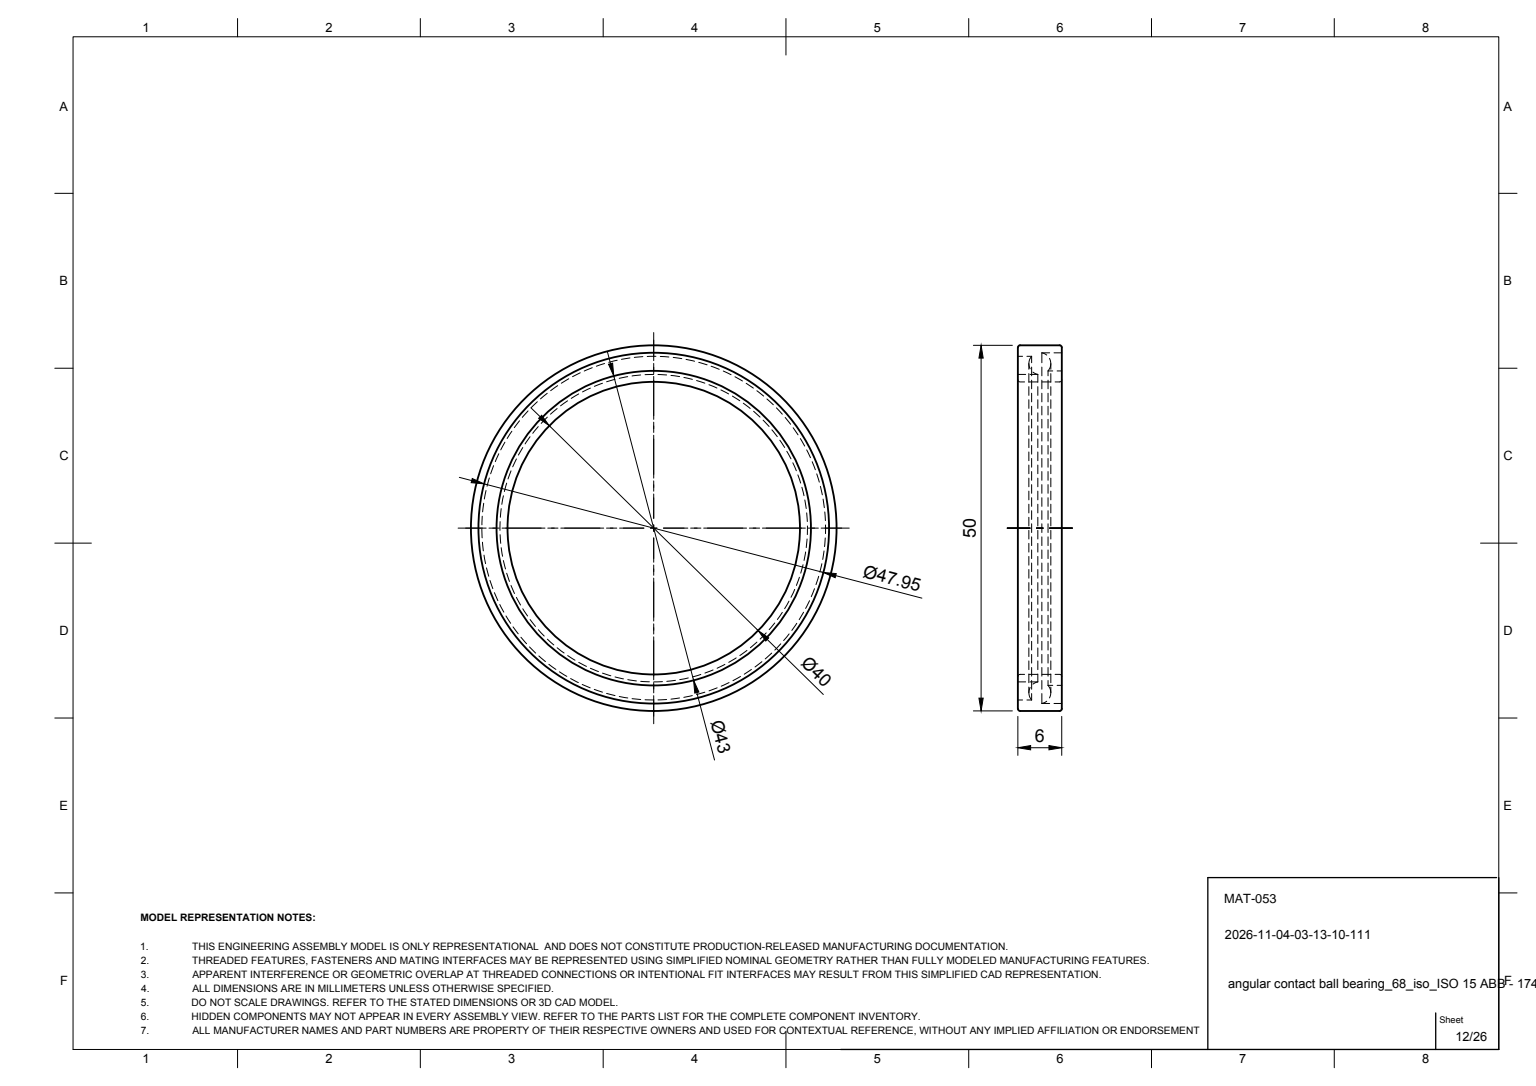
ISO-10303-21;
HEADER;
FILE_DESCRIPTION (('STEP AP214'),
    '1' );
FILE_NAME ('angular contact ball bearing_68_iso_ISO 15 ABB - 1740 - 38,SI,NC,38_68.step',
    '2026-10-10T03:43:58',
    ( '' ),
    ( '' ),
    'SwSTEP 2.0',
    'SolidWorks 2026',
    '' );
FILE_SCHEMA (( 'AUTOMOTIVE_DESIGN' ));
ENDSEC;

DATA;
#280=CARTESIAN_POINT ( 'NONE',  ( -20.63749999999999574, 0.000000000000000000, 0.000000000000000000 ) ) ;
#290=CYLINDRICAL_SURFACE ( 'NONE', #39876, 21.02500000000000213 ) ;
#373=EDGE_CURVE ( 'NONE', #61321, #29458, #45223, .T. ) ;
#397=AXIS2_PLACEMENT_3D ( 'NONE', #30126, #55451, #24841 ) ;
#538=EDGE_CURVE ( 'NONE', #52559, #9895, #28349, .T. ) ;
#593=CARTESIAN_POINT ( 'NONE',  ( 3.000000000000002665, 0.000000000000000000, 0.000000000000000000 ) ) ;
#621=( GEOMETRIC_REPRESENTATION_CONTEXT ( 3 ) GLOBAL_UNCERTAINTY_ASSIGNED_CONTEXT ( ( #45151 ) ) GLOBAL_UNIT_ASSIGNED_CONTEXT ( ( #57453, #30034, #6044 ) ) REPRESENTATION_CONTEXT ( 'NONE', 'WORKASPACE' ) );
#645=DIRECTION ( 'NONE',  ( -1.000000000000000000, -0.000000000000000000, -0.000000000000000000 ) ) ;
#660=AXIS2_PLACEMENT_3D ( 'NONE', #33851, #12745, #56006 ) ;
#969=CIRCLE ( 'NONE', #42531, 0.3000000000000051514 ) ;
#1025=DIRECTION ( 'NONE',  ( -0.000000000000000000, 0.000000000000000000, 1.000000000000000000 ) ) ;
#1055=EDGE_LOOP ( 'NONE', ( #53256, #11888, #11752, #31216 ) ) ;
#1105=CARTESIAN_POINT ( 'NONE',  ( -20.63749999999999929, 2.574819895207310592E-15, 21.02500000000000213 ) ) ;
#1307=EDGE_LOOP ( 'NONE', ( #35299, #10153, #10005, #63339 ) ) ;
#1323=TOROIDAL_SURFACE ( 'NONE', #20399, 22.50000000000000000, 1.500000000000000444 ) ;
#1417=AXIS2_PLACEMENT_3D ( 'NONE', #30152, #18895, #57567 ) ;
#1469=SURFACE_SIDE_STYLE ('',( #55275 ) ) ;
#1536=CARTESIAN_POINT ( 'NONE',  ( 3.000000000000006217, 0.000000000000000000, 0.000000000000000000 ) ) ;
#1545=ORIENTED_EDGE ( 'NONE', *, *, #39490, .T. ) ;
#1648=FACE_OUTER_BOUND ( 'NONE', #49556, .T. ) ;
#1676=AXIS2_PLACEMENT_3D ( 'NONE', #6098, #53928, #48643 ) ;
#1879=CIRCLE ( 'NONE', #29940, 1.500000000000001332 ) ;
#1883=DIRECTION ( 'NONE',  ( 0.000000000000000000, 0.000000000000000000, -1.000000000000000000 ) ) ;
#1943=CARTESIAN_POINT ( 'NONE',  ( -0.2727178028659107967, 2.936090700955778964E-15, -23.97499999999999787 ) ) ;
#1945=ORIENTED_EDGE ( 'NONE', *, *, #538, .F. ) ;
#2038=CIRCLE ( 'NONE', #53667, 25.00000000000000355 ) ;
#2107=ORIENTED_EDGE ( 'NONE', *, *, #62169, .F. ) ;
#2116=DIRECTION ( 'NONE',  ( 1.000000000000000000, 0.000000000000000000, 0.000000000000000000 ) ) ;
#2288=DIRECTION ( 'NONE',  ( -0.000000000000000000, 0.000000000000000000, 1.000000000000000000 ) ) ;
#2314=ORIENTED_EDGE ( 'NONE', *, *, #36138, .T. ) ;
#2373=DIRECTION ( 'NONE',  ( 1.000000000000000000, 0.000000000000000000, 0.000000000000000000 ) ) ;
#2396=MECHANICAL_DESIGN_GEOMETRIC_PRESENTATION_REPRESENTATION('',(#32715),#59658);
#2447=CYLINDRICAL_SURFACE ( 'NONE', #33618, 25.00000000000000711 ) ;
#2492=DIRECTION ( 'NONE',  ( 0.000000000000000000, -1.000000000000000000, 0.000000000000000000 ) ) ;
#2692=CARTESIAN_POINT ( 'NONE',  ( 2.699999999999990408, 0.000000000000000000, 0.000000000000000000 ) ) ;
#2799=ADVANCED_FACE ( 'NONE', ( #20237 ), #8332, .T. ) ;
#2890=LINE ( 'NONE', #34569, #25833 ) ;
#2981=EDGE_LOOP ( 'NONE', ( #13147, #27199, #10225, #40250 ) ) ;
#3058=EDGE_CURVE ( 'NONE', #60812, #57773, #58704, .T. ) ;
#3118=CARTESIAN_POINT ( 'NONE',  ( 2.999999999999992450, 0.000000000000000000, 0.000000000000000000 ) ) ;
#3137=DIRECTION ( 'NONE',  ( 1.000000000000000000, 0.000000000000000000, 0.000000000000000000 ) ) ;
#3249=EDGE_LOOP ( 'NONE', ( #58804, #53989, #66441, #9980 ) ) ;
#3441=DIRECTION ( 'NONE',  ( 0.000000000000000000, 0.000000000000000000, -1.000000000000000000 ) ) ;
#3503=CIRCLE ( 'NONE', #56271, 24.69999999999999929 ) ;
#3556=DIRECTION ( 'NONE',  ( 1.000000000000000000, 0.000000000000000000, 0.000000000000000000 ) ) ;
#3565=DIRECTION ( 'NONE',  ( -1.000000000000000000, -0.000000000000000000, -0.000000000000000000 ) ) ;
#3692=AXIS2_PLACEMENT_3D ( 'NONE', #33582, #55008, #6830 ) ;
#3738=ORIENTED_EDGE ( 'NONE', *, *, #14434, .T. ) ;
#3880=EDGE_CURVE ( 'NONE', #19652, #60812, #44141, .T. ) ;
#4000=AXIS2_PLACEMENT_3D ( 'NONE', #32142, #21921, #69063 ) ;
#4007=CYLINDRICAL_SURFACE ( 'NONE', #6388, 23.50000000000000000 ) ;
#4031=AXIS2_PLACEMENT_3D ( 'NONE', #27744, #49185, #1025 ) ;
#4149=CIRCLE ( 'NONE', #55822, 1.500000000000001332 ) ;
#4152=ADVANCED_FACE ( 'NONE', ( #15588, #58822 ), #37037, .T. ) ;
#4194=ORIENTED_EDGE ( 'NONE', *, *, #40811, .F. ) ;
#4257=VERTEX_POINT ( 'NONE', #31338 ) ;
#4325=DIRECTION ( 'NONE',  ( 1.000000000000000000, 0.000000000000000000, 0.000000000000000000 ) ) ;
#4352=FACE_OUTER_BOUND ( 'NONE', #11897, .T. ) ;
#4484=EDGE_LOOP ( 'NONE', ( #2107, #34781, #40469, #13611 ) ) ;
#4509=AXIS2_PLACEMENT_3D ( 'NONE', #52504, #4325, #66976 ) ;
#4534=CARTESIAN_POINT ( 'NONE',  ( 2.699999999999990408, 2.467663300281916154E-15, 19.99999999999998934 ) ) ;
#4593=PRODUCT_DEFINITION_SHAPE ( 'NONE', 'NONE',  #56848 ) ;
#4670=DIRECTION ( 'NONE',  ( 0.000000000000000000, 0.000000000000000000, -1.000000000000000000 ) ) ;
#4680=CARTESIAN_POINT ( 'NONE',  ( -2.699999999999990408, 0.000000000000000000, 0.000000000000000000 ) ) ;
#4739=AXIS2_PLACEMENT_3D ( 'NONE', #280, #64310, #58676 ) ;
#4831=VECTOR ( 'NONE', #25004, 1000.000000000000000 ) ;
#5355=EDGE_LOOP ( 'NONE', ( #29578, #35095, #48562, #52524 ) ) ;
#5423=ORIENTED_EDGE ( 'NONE', *, *, #38504, .T. ) ;
#5446=DIRECTION ( 'NONE',  ( 1.000000000000000000, 0.000000000000000000, 0.000000000000000000 ) ) ;
#5645=EDGE_CURVE ( 'NONE', #52559, #6514, #31915, .T. ) ;
#5676=AXIS2_PLACEMENT_3D ( 'NONE', #13153, #67320, #40560 ) ;
#5689=PRESENTATION_STYLE_ASSIGNMENT (( #49641 ) ) ;
#5737=DIRECTION ( 'NONE',  ( 0.000000000000000000, 0.000000000000000000, -1.000000000000000000 ) ) ;
#6044=( NAMED_UNIT ( * ) SI_UNIT ( $, .STERADIAN. ) SOLID_ANGLE_UNIT ( ) );
#6069=TOROIDAL_SURFACE ( 'NONE', #61121, 20.30000000000000071, 0.3000000000000062061 ) ;
#6074=CIRCLE ( 'NONE', #45411, 0.3000000000000051514 ) ;
#6098=CARTESIAN_POINT ( 'NONE',  ( -2.699999999999990408, 0.000000000000000000, 0.000000000000000000 ) ) ;
#6152=ORIENTED_EDGE ( 'NONE', *, *, #29172, .T. ) ;
#6170=AXIS2_PLACEMENT_3D ( 'NONE', #8294, #46253, #41679 ) ;
#6245=DIRECTION ( 'NONE',  ( 0.000000000000000000, 1.000000000000000000, -1.224646799147353207E-16 ) ) ;
#6250=DIRECTION ( 'NONE',  ( 0.000000000000000000, 0.000000000000000000, -1.000000000000000000 ) ) ;
#6260=CARTESIAN_POINT ( 'NONE',  ( 0.2727178028659107412, 0.000000000000000000, 0.000000000000000000 ) ) ;
#6278=DIRECTION ( 'NONE',  ( 0.000000000000000000, 1.000000000000000000, -1.224646799147353207E-16 ) ) ;
#6294=FACE_OUTER_BOUND ( 'NONE', #48770, .T. ) ;
#6341=EDGE_CURVE ( 'NONE', #42528, #57773, #66837, .T. ) ;
#6372=DIRECTION ( 'NONE',  ( 1.000000000000000000, 0.000000000000000000, 0.000000000000000000 ) ) ;
#6388=AXIS2_PLACEMENT_3D ( 'NONE', #14557, #51162, #19139 ) ;
#6392=CIRCLE ( 'NONE', #41248, 23.97499999999999787 ) ;
#6514=VERTEX_POINT ( 'NONE', #4534 ) ;
#6524=CARTESIAN_POINT ( 'NONE',  ( 0.2727178028659107412, 0.000000000000000000, 21.02500000000000213 ) ) ;
#6527=EDGE_LOOP ( 'NONE', ( #17045, #8583, #48179, #6821 ) ) ;
#6821=ORIENTED_EDGE ( 'NONE', *, *, #45518, .F. ) ;
#6830=DIRECTION ( 'NONE',  ( 0.000000000000000000, -1.224646799147351975E-16, 1.000000000000000000 ) ) ;
#6953=DIRECTION ( 'NONE',  ( -1.000000000000000000, -0.000000000000000000, -0.000000000000000000 ) ) ;
#7109=AXIS2_PLACEMENT_3D ( 'NONE', #17385, #52177, #56771 ) ;
#7160=ORIENTED_EDGE ( 'NONE', *, *, #39490, .F. ) ;
#7202=DIRECTION ( 'NONE',  ( 1.000000000000000000, 0.000000000000000000, 0.000000000000000000 ) ) ;
#7301=CIRCLE ( 'NONE', #6170, 23.97499999999999787 ) ;
#7431=DIRECTION ( 'NONE',  ( 0.000000000000000000, 0.000000000000000000, -1.000000000000000000 ) ) ;
#7736=DIRECTION ( 'NONE',  ( 0.000000000000000000, 0.000000000000000000, 1.000000000000000000 ) ) ;
#7907=ORIENTED_EDGE ( 'NONE', *, *, #42027, .T. ) ;
#7941=ORIENTED_EDGE ( 'NONE', *, *, #41756, .F. ) ;
#8069=LINE ( 'NONE', #52019, #34673 ) ;
#8081=ORIENTED_EDGE ( 'NONE', *, *, #9301, .F. ) ;
#8105=CIRCLE ( 'NONE', #49656, 0.3000000000000051514 ) ;
#8217=FACE_OUTER_BOUND ( 'NONE', #67323, .T. ) ;
#8282=ORIENTED_EDGE ( 'NONE', *, *, #373, .T. ) ;
#8294=CARTESIAN_POINT ( 'NONE',  ( -3.000000000000006217, 0.000000000000000000, 0.000000000000000000 ) ) ;
#8299=CARTESIAN_POINT ( 'NONE',  ( 3.000000000000002665, 0.000000000000000000, 0.000000000000000000 ) ) ;
#8307=FACE_OUTER_BOUND ( 'NONE', #58252, .T. ) ;
#8319=DIRECTION ( 'NONE',  ( 1.000000000000000000, 0.000000000000000000, 0.000000000000000000 ) ) ;
#8332=TOROIDAL_SURFACE ( 'NONE', #38593, 22.50000000000000000, 1.500000000000000444 ) ;
#8508=CIRCLE ( 'NONE', #25338, 23.50000000000000000 ) ;
#8570=FACE_BOUND ( 'NONE', #68279, .T. ) ;
#8583=ORIENTED_EDGE ( 'NONE', *, *, #38351, .T. ) ;
#8602=FACE_OUTER_BOUND ( 'NONE', #58165, .T. ) ;
#8641=FACE_OUTER_BOUND ( 'NONE', #30628, .T. ) ;
#8658=DIRECTION ( 'NONE',  ( 1.000000000000000000, 0.000000000000000000, 0.000000000000000000 ) ) ;
#8689=ORIENTED_EDGE ( 'NONE', *, *, #38093, .T. ) ;
#8731=CARTESIAN_POINT ( 'NONE',  ( 0.000000000000000000, 0.000000000000000000, 22.50000000000000000 ) ) ;
#8749=DIRECTION ( 'NONE',  ( 0.000000000000000000, 0.000000000000000000, -1.000000000000000000 ) ) ;
#8764=CARTESIAN_POINT ( 'NONE',  ( 2.699999999999990408, 0.000000000000000000, -20.30000000000000071 ) ) ;
#8768=EDGE_CURVE ( 'NONE', #9895, #52559, #26535, .T. ) ;
#8902=ORIENTED_EDGE ( 'NONE', *, *, #22144, .F. ) ;
#8954=DIRECTION ( 'NONE',  ( 1.000000000000000000, 0.000000000000000000, 0.000000000000000000 ) ) ;
#8961=EDGE_CURVE ( 'NONE', #25778, #4257, #37775, .T. ) ;
#8982=DIRECTION ( 'NONE',  ( 0.000000000000000000, 0.000000000000000000, -1.000000000000000000 ) ) ;
#8995=DIRECTION ( 'NONE',  ( 0.000000000000000000, 0.000000000000000000, -1.000000000000000000 ) ) ;
#9009=EDGE_CURVE ( 'NONE', #33511, #39615, #42211, .T. ) ;
#9167=ORIENTED_EDGE ( 'NONE', *, *, #64153, .T. ) ;
#9281=CARTESIAN_POINT ( 'NONE',  ( -2.999999999999990674, 21.50000000000000000, 0.000000000000000000 ) ) ;
#9301=EDGE_CURVE ( 'NONE', #61321, #61115, #4149, .T. ) ;
#9888=ORIENTED_EDGE ( 'NONE', *, *, #67535, .T. ) ;
#9895=VERTEX_POINT ( 'NONE', #49076 ) ;
#9905=EDGE_LOOP ( 'NONE', ( #64861, #51171, #32704, #4194 ) ) ;
#9922=CARTESIAN_POINT ( 'NONE',  ( -3.000000000000002665, 0.000000000000000000, 0.000000000000000000 ) ) ;
#9980=ORIENTED_EDGE ( 'NONE', *, *, #39856, .F. ) ;
#10005=ORIENTED_EDGE ( 'NONE', *, *, #45518, .T. ) ;
#10153=ORIENTED_EDGE ( 'NONE', *, *, #15775, .T. ) ;
#10169=AXIS2_PLACEMENT_3D ( 'NONE', #18519, #39968, #29417 ) ;
#10225=ORIENTED_EDGE ( 'NONE', *, *, #65595, .T. ) ;
#10277=FILL_AREA_STYLE ('',( #48241 ) ) ;
#10671=FACE_OUTER_BOUND ( 'NONE', #1307, .T. ) ;
#10835=CARTESIAN_POINT ( 'NONE',  ( -0.2727178028659107412, 0.000000000000000000, 0.000000000000000000 ) ) ;
#10895=VECTOR ( 'NONE', #8954, 1000.000000000000000 ) ;
#10939=CARTESIAN_POINT ( 'NONE',  ( 2.700000000000004619, 0.000000000000000000, -24.69999999999999929 ) ) ;
#11062=DIRECTION ( 'NONE',  ( 0.000000000000000000, 0.000000000000000000, -1.000000000000000000 ) ) ;
#11493=CARTESIAN_POINT ( 'NONE',  ( -3.000000000000002665, 0.000000000000000000, -24.69999999999999929 ) ) ;
#11592=CARTESIAN_POINT ( 'NONE',  ( -2.699999999999990408, 0.000000000000000000, 0.000000000000000000 ) ) ;
#11700=EDGE_LOOP ( 'NONE', ( #28380, #69331, #41144, #54488 ) ) ;
#11752=ORIENTED_EDGE ( 'NONE', *, *, #36138, .F. ) ;
#11888=ORIENTED_EDGE ( 'NONE', *, *, #36705, .T. ) ;
#11897=EDGE_LOOP ( 'NONE', ( #34288, #67277, #15013, #55475 ) ) ;
#11898=AXIS2_PLACEMENT_3D ( 'NONE', #593, #21349, #64613 ) ;
#12131=CARTESIAN_POINT ( 'NONE',  ( -20.63749999999999574, 0.000000000000000000, 0.000000000000000000 ) ) ;
#12172=CYLINDRICAL_SURFACE ( 'NONE', #65307, 23.97499999999999787 ) ;
#12227=EDGE_CURVE ( 'NONE', #27706, #49790, #6392, .T. ) ;
#12368=ORIENTED_EDGE ( 'NONE', *, *, #23031, .T. ) ;
#12612=LINE ( 'NONE', #24216, #42663 ) ;
#12629=AXIS2_PLACEMENT_3D ( 'NONE', #11592, #33073, #54500 ) ;
#12745=DIRECTION ( 'NONE',  ( 1.000000000000000000, 0.000000000000000000, 0.000000000000000000 ) ) ;
#13006=ORIENTED_EDGE ( 'NONE', *, *, #22230, .T. ) ;
#13147=ORIENTED_EDGE ( 'NONE', *, *, #67535, .F. ) ;
#13153=CARTESIAN_POINT ( 'NONE',  ( -2.999999999999992450, 0.000000000000000000, 0.000000000000000000 ) ) ;
#13239=ORIENTED_EDGE ( 'NONE', *, *, #538, .T. ) ;
#13285=CARTESIAN_POINT ( 'NONE',  ( -2.999999999999994227, 2.486033002269127373E-15, 20.30000000000000071 ) ) ;
#13313=DIRECTION ( 'NONE',  ( 0.000000000000000000, -1.000000000000000000, 0.000000000000000000 ) ) ;
#13420=DIRECTION ( 'NONE',  ( 0.000000000000000000, 0.000000000000000000, -1.000000000000000000 ) ) ;
#13611=ORIENTED_EDGE ( 'NONE', *, *, #42027, .F. ) ;
#13832=PLANE ( 'NONE',  #4509 ) ;
#13977=EDGE_CURVE ( 'NONE', #25778, #55030, #12612, .T. ) ;
#14023=DIRECTION ( 'NONE',  ( 0.000000000000000000, 0.000000000000000000, -1.000000000000000000 ) ) ;
#14189=EDGE_LOOP ( 'NONE', ( #68269, #54237, #67546, #12368 ) ) ;
#14234=CARTESIAN_POINT ( 'NONE',  ( -20.63749999999999929, 0.000000000000000000, 0.000000000000000000 ) ) ;
#14434=EDGE_CURVE ( 'NONE', #51018, #67247, #22479, .T. ) ;
#14557=CARTESIAN_POINT ( 'NONE',  ( -20.63749999999999574, 0.000000000000000000, 0.000000000000000000 ) ) ;
#14649=FACE_OUTER_BOUND ( 'NONE', #6527, .T. ) ;
#14664=CARTESIAN_POINT ( 'NONE',  ( 1.118033988749894458, 0.000000000000000000, 23.50000000000000000 ) ) ;
#14748=ADVANCED_FACE ( 'NONE', ( #8217, #8570 ), #13832, .T. ) ;
#14827=AXIS2_PLACEMENT_3D ( 'NONE', #34032, #29103, #66407 ) ;
#15013=ORIENTED_EDGE ( 'NONE', *, *, #51063, .T. ) ;
#15387=EDGE_CURVE ( 'NONE', #19256, #46466, #30421, .T. ) ;
#15483=DIRECTION ( 'NONE',  ( 1.000000000000000000, 0.000000000000000000, 0.000000000000000000 ) ) ;
#15588=FACE_OUTER_BOUND ( 'NONE', #24203, .T. ) ;
#15589=CARTESIAN_POINT ( 'NONE',  ( 3.000000000000006217, 2.877919977996280320E-15, 23.50000000000000000 ) ) ;
#15676=CARTESIAN_POINT ( 'NONE',  ( -1.118033988749894458, 0.000000000000000000, -21.50000000000000000 ) ) ;
#15775=EDGE_CURVE ( 'NONE', #44335, #54364, #3503, .T. ) ;
#16011=ORIENTED_EDGE ( 'NONE', *, *, #65424, .F. ) ;
#16224=DIRECTION ( 'NONE',  ( 0.000000000000000000, 0.000000000000000000, -1.000000000000000000 ) ) ;
#16263=CARTESIAN_POINT ( 'NONE',  ( 3.000000000000003997, 24.69999999999999929, 0.000000000000000000 ) ) ;
#16286=LINE ( 'NONE', #27882, #17334 ) ;
#16318=AXIS2_PLACEMENT_3D ( 'NONE', #14234, #18814, #68051 ) ;
#16344=CARTESIAN_POINT ( 'NONE',  ( -1.118033988749894458, 2.632990618166809235E-15, 21.50000000000000000 ) ) ;
#16665=AXIS2_PLACEMENT_3D ( 'NONE', #47766, #21050, #42497 ) ;
#16734=FACE_OUTER_BOUND ( 'NONE', #46287, .T. ) ;
#16810=VECTOR ( 'NONE', #52108, 1000.000000000000000 ) ;
#16904=ORIENTED_EDGE ( 'NONE', *, *, #31935, .F. ) ;
#17034=DIRECTION ( 'NONE',  ( 1.000000000000000000, 0.000000000000000000, 0.000000000000000000 ) ) ;
#17045=ORIENTED_EDGE ( 'NONE', *, *, #61298, .T. ) ;
#17193=ORIENTED_EDGE ( 'NONE', *, *, #64153, .F. ) ;
#17319=EDGE_LOOP ( 'NONE', ( #16011, #64545, #1545, #18990 ) ) ;
#17334=VECTOR ( 'NONE', #54952, 1000.000000000000000 ) ;
#17385=CARTESIAN_POINT ( 'NONE',  ( 0.2727178028659107412, 0.000000000000000000, 0.000000000000000000 ) ) ;
#17532=DIRECTION ( 'NONE',  ( 1.000000000000000000, 0.000000000000000000, 0.000000000000000000 ) ) ;
#17543=DIRECTION ( 'NONE',  ( 1.000000000000000000, 0.000000000000000000, 0.000000000000000000 ) ) ;
#17547=PLANE ( 'NONE',  #4031 ) ;
#17567=MANIFOLD_SOLID_BREP ( 'OuterRace', #41822 ) ;
#17705=DIRECTION ( 'NONE',  ( 1.000000000000000000, 0.000000000000000000, 0.000000000000000000 ) ) ;
#17843=AXIS2_PLACEMENT_3D ( 'NONE', #23168, #60786, #23518 ) ;
#17861=VERTEX_POINT ( 'NONE', #39721 ) ;
#17880=ORIENTED_EDGE ( 'NONE', *, *, #15387, .T. ) ;
#18211=TOROIDAL_SURFACE ( 'NONE', #14827, 22.50000000000000000, 1.500000000000000444 ) ;
#18246=AXIS2_PLACEMENT_3D ( 'NONE', #29107, #2373, #23830 ) ;
#18277=CARTESIAN_POINT ( 'NONE',  ( -20.63749999999999574, 0.000000000000000000, 0.000000000000000000 ) ) ;
#18384=CIRCLE ( 'NONE', #22907, 23.97499999999999787 ) ;
#18451=ADVANCED_FACE ( 'NONE', ( #54411 ), #18211, .T. ) ;
#18519=CARTESIAN_POINT ( 'NONE',  ( -2.999999999999992450, 0.000000000000000000, 0.000000000000000000 ) ) ;
#18814=DIRECTION ( 'NONE',  ( 1.000000000000000000, 0.000000000000000000, 0.000000000000000000 ) ) ;
#18895=DIRECTION ( 'NONE',  ( 1.000000000000000000, 0.000000000000000000, 0.000000000000000000 ) ) ;
#18903=ADVANCED_FACE ( 'NONE', ( #24777, #25130 ), #46563, .T. ) ;
#18946=CARTESIAN_POINT ( 'NONE',  ( -3.000000000000006217, 0.000000000000000000, 0.000000000000000000 ) ) ;
#18974=EDGE_LOOP ( 'NONE', ( #53039, #30160, #8689, #23492 ) ) ;
#18990=ORIENTED_EDGE ( 'NONE', *, *, #41756, .T. ) ;
#19103=CIRCLE ( 'NONE', #65146, 25.00000000000000355 ) ;
#19139=DIRECTION ( 'NONE',  ( 0.000000000000000000, 0.000000000000000000, -1.000000000000000000 ) ) ;
#19240=APPLICATION_CONTEXT ( 'automotive_design' ) ;
#19256=VERTEX_POINT ( 'NONE', #13285 ) ;
#19482=ORIENTED_EDGE ( 'NONE', *, *, #21650, .F. ) ;
#19561=DIRECTION ( 'NONE',  ( 0.000000000000000000, 0.000000000000000000, -1.000000000000000000 ) ) ;
#19652=VERTEX_POINT ( 'NONE', #6524 ) ;
#19854=FACE_OUTER_BOUND ( 'NONE', #27189, .T. ) ;
#20081=ORIENTED_EDGE ( 'NONE', *, *, #29172, .F. ) ;
#20183=EDGE_LOOP ( 'NONE', ( #2314, #17880 ) ) ;
#20189=LINE ( 'NONE', #63102, #10895 ) ;
#20237=FACE_OUTER_BOUND ( 'NONE', #26458, .T. ) ;
#20353=AXIS2_PLACEMENT_3D ( 'NONE', #12131, #17034, #49392 ) ;
#20399=AXIS2_PLACEMENT_3D ( 'NONE', #68953, #3565, #29959 ) ;
#20565=DIRECTION ( 'NONE',  ( 1.000000000000000000, 0.000000000000000000, 0.000000000000000000 ) ) ;
#20645=AXIS2_PLACEMENT_3D ( 'NONE', #23971, #66903, #13420 ) ;
#21001=CIRCLE ( 'NONE', #38941, 24.69999999999999929 ) ;
#21010=EDGE_LOOP ( 'NONE', ( #22173, #19482 ) ) ;
#21050=DIRECTION ( 'NONE',  ( 1.000000000000000000, 0.000000000000000000, 0.000000000000000000 ) ) ;
#21349=DIRECTION ( 'NONE',  ( 1.000000000000000000, 0.000000000000000000, 0.000000000000000000 ) ) ;
#21574=FACE_OUTER_BOUND ( 'NONE', #11700, .T. ) ;
#21650=EDGE_CURVE ( 'NONE', #31540, #33414, #63244, .T. ) ;
#21803=CARTESIAN_POINT ( 'NONE',  ( -2.999999999999992450, 2.632990618166809235E-15, 21.50000000000000000 ) ) ;
#21921=DIRECTION ( 'NONE',  ( 1.000000000000000000, 0.000000000000000000, 0.000000000000000000 ) ) ;
#22144=EDGE_CURVE ( 'NONE', #17861, #66051, #63291, .T. ) ;
#22173=ORIENTED_EDGE ( 'NONE', *, *, #29173, .F. ) ;
#22230=EDGE_CURVE ( 'NONE', #4257, #6514, #41435, .T. ) ;
#22432=LINE ( 'NONE', #36973, #16810 ) ;
#22479=CIRCLE ( 'NONE', #35995, 24.69999999999999929 ) ;
#22853=AXIS2_PLACEMENT_3D ( 'NONE', #64535, #5446, #11062 ) ;
#22907=AXIS2_PLACEMENT_3D ( 'NONE', #33174, #60245, #45104 ) ;
#23007=AXIS2_PLACEMENT_3D ( 'NONE', #68736, #63132, #8982 ) ;
#23031=EDGE_CURVE ( 'NONE', #55030, #6514, #28543, .T. ) ;
#23168=CARTESIAN_POINT ( 'NONE',  ( 2.699999999999990408, 0.000000000000000000, 0.000000000000000000 ) ) ;
#23260=CARTESIAN_POINT ( 'NONE',  ( -2.700000000000004619, 0.000000000000000000, -24.69999999999999929 ) ) ;
#23340=ORIENTED_EDGE ( 'NONE', *, *, #29173, .T. ) ;
#23492=ORIENTED_EDGE ( 'NONE', *, *, #45920, .F. ) ;
#23518=DIRECTION ( 'NONE',  ( 0.000000000000000000, 0.000000000000000000, -1.000000000000000000 ) ) ;
#23576=EDGE_CURVE ( 'NONE', #31797, #67247, #6074, .T. ) ;
#23614=LINE ( 'NONE', #34528, #4831 ) ;
#23830=DIRECTION ( 'NONE',  ( 0.000000000000000000, 0.000000000000000000, -1.000000000000000000 ) ) ;
#23960=ADVANCED_FACE ( 'NONE', ( #1648 ), #40996, .T. ) ;
#23971=CARTESIAN_POINT ( 'NONE',  ( 2.699999999999990408, 0.000000000000000000, 0.000000000000000000 ) ) ;
#23978=AXIS2_PLACEMENT_3D ( 'NONE', #46257, #61744, #25523 ) ;
#24203=EDGE_LOOP ( 'NONE', ( #51317, #3738 ) ) ;
#24216=CARTESIAN_POINT ( 'NONE',  ( -20.63749999999999929, 0.000000000000000000, -19.99999999999999289 ) ) ;
#24261=DIRECTION ( 'NONE',  ( 0.000000000000000000, 0.000000000000000000, -1.000000000000000000 ) ) ;
#24277=ORIENTED_EDGE ( 'NONE', *, *, #15775, .F. ) ;
#24286=CARTESIAN_POINT ( 'NONE',  ( 0.000000000000000000, 2.755455298081544778E-15, -22.50000000000000000 ) ) ;
#24770=DIRECTION ( 'NONE',  ( 0.000000000000000000, 0.000000000000000000, -1.000000000000000000 ) ) ;
#24777=FACE_BOUND ( 'NONE', #20183, .T. ) ;
#24841=DIRECTION ( 'NONE',  ( 0.000000000000000000, 0.000000000000000000, -1.000000000000000000 ) ) ;
#24845=FACE_OUTER_BOUND ( 'NONE', #3249, .T. ) ;
#24885=CIRCLE ( 'NONE', #27067, 0.3000000000000051514 ) ;
#24957=CARTESIAN_POINT ( 'NONE',  ( -3.000000000000006217, 2.936090700955778569E-15, 23.97499999999999787 ) ) ;
#25004=DIRECTION ( 'NONE',  ( 1.000000000000000000, 0.000000000000000000, 0.000000000000000000 ) ) ;
#25130=FACE_OUTER_BOUND ( 'NONE', #21010, .T. ) ;
#25190=ADVANCED_FACE ( 'NONE', ( #4352 ), #60157, .T. ) ;
#25281=CARTESIAN_POINT ( 'NONE',  ( -2.700000000000004619, 0.000000000000000000, -25.00000000000000711 ) ) ;
#25338=AXIS2_PLACEMENT_3D ( 'NONE', #1536, #44081, #33566 ) ;
#25450=ORIENTED_EDGE ( 'NONE', *, *, #49938, .F. ) ;
#25456=UNCERTAINTY_MEASURE_WITH_UNIT (LENGTH_MEASURE( 1.000000000000000082E-05 ), #48934, 'distance_accuracy_value', 'NONE');
#25517=ADVANCED_FACE ( 'NONE', ( #55292 ), #55642, .T. ) ;
#25523=DIRECTION ( 'NONE',  ( 0.000000000000000000, 0.000000000000000000, -1.000000000000000000 ) ) ;
#25778=VERTEX_POINT ( 'NONE', #59093 ) ;
#25833=VECTOR ( 'NONE', #61281, 1000.000000000000000 ) ;
#25907=DIRECTION ( 'NONE',  ( 0.000000000000000000, 1.224646799147357891E-16, 1.000000000000000000 ) ) ;
#25930=EDGE_LOOP ( 'NONE', ( #58701, #62122 ) ) ;
#26146=DIRECTION ( 'NONE',  ( 1.000000000000000000, 0.000000000000000000, 0.000000000000000000 ) ) ;
#26234=VECTOR ( 'NONE', #51646, 1000.000000000000000 ) ;
#26458=EDGE_LOOP ( 'NONE', ( #42578, #31480, #34661, #36762 ) ) ;
#26510=PRODUCT ( 'angular contact ball bearing_68_iso_ISO 15 ABB - 1740 - 38,SI,NC,38_68', 'angular contact ball bearing_68_iso_ISO 15 ABB - 1740 - 38,SI,NC,38_68', '', ( #36097 ) ) ;
#26535=CIRCLE ( 'NONE', #42303, 20.30000000000000071 ) ;
#26670=DIRECTION ( 'NONE',  ( 0.000000000000000000, 0.000000000000000000, -1.000000000000000000 ) ) ;
#27067=AXIS2_PLACEMENT_3D ( 'NONE', #61611, #38772, #60565 ) ;
#27077=AXIS2_PLACEMENT_3D ( 'NONE', #65906, #17705, #1883 ) ;
#27133=CARTESIAN_POINT ( 'NONE',  ( -20.63749999999999574, 0.000000000000000000, -23.50000000000000000 ) ) ;
#27150=EDGE_CURVE ( 'NONE', #49790, #27706, #7301, .T. ) ;
#27189=EDGE_LOOP ( 'NONE', ( #61034, #13006, #9167, #32258 ) ) ;
#27199=ORIENTED_EDGE ( 'NONE', *, *, #67117, .F. ) ;
#27347=CARTESIAN_POINT ( 'NONE',  ( -2.700000000000004619, 3.024877593893962577E-15, 24.69999999999999929 ) ) ;
#27397=EDGE_CURVE ( 'NONE', #60665, #30714, #8508, .T. ) ;
#27450=TOROIDAL_SURFACE ( 'NONE', #51081, 22.50000000000000000, 1.500000000000000444 ) ;
#27706=VERTEX_POINT ( 'NONE', #40473 ) ;
#27744=CARTESIAN_POINT ( 'NONE',  ( -3.000000000000003997, 23.97499999999999787, 0.000000000000000000 ) ) ;
#27882=CARTESIAN_POINT ( 'NONE',  ( -20.63749999999999929, 0.000000000000000000, -21.50000000000000000 ) ) ;
#27951=CYLINDRICAL_SURFACE ( 'NONE', #20353, 23.97499999999999787 ) ;
#28025=ADVANCED_FACE ( 'NONE', ( #54462, #6294 ), #17547, .T. ) ;
#28105=DIRECTION ( 'NONE',  ( 1.000000000000000000, 0.000000000000000000, 0.000000000000000000 ) ) ;
#28349=CIRCLE ( 'NONE', #29461, 20.30000000000000071 ) ;
#28380=ORIENTED_EDGE ( 'NONE', *, *, #34961, .T. ) ;
#28417=EDGE_CURVE ( 'NONE', #67247, #51018, #69191, .T. ) ;
#28479=TOROIDAL_SURFACE ( 'NONE', #397, 24.69999999999999929, 0.3000000000000035971 ) ;
#28543=CIRCLE ( 'NONE', #20645, 19.99999999999998934 ) ;
#28562=CARTESIAN_POINT ( 'NONE',  ( 3.000000000000006217, 0.000000000000000000, 0.000000000000000000 ) ) ;
#28662=DIRECTION ( 'NONE',  ( 0.000000000000000000, 0.000000000000000000, -1.000000000000000000 ) ) ;
#28700=TOROIDAL_SURFACE ( 'NONE', #4000, 24.69999999999999929, 0.3000000000000035971 ) ;
#28962=CARTESIAN_POINT ( 'NONE',  ( 2.700000000000004619, 0.000000000000000000, 0.000000000000000000 ) ) ;
#29103=DIRECTION ( 'NONE',  ( -1.000000000000000000, -0.000000000000000000, -0.000000000000000000 ) ) ;
#29107=CARTESIAN_POINT ( 'NONE',  ( -2.700000000000004619, 0.000000000000000000, 0.000000000000000000 ) ) ;
#29172=EDGE_CURVE ( 'NONE', #9895, #55030, #45658, .T. ) ;
#29173=EDGE_CURVE ( 'NONE', #33414, #31540, #47897, .T. ) ;
#29206=DIRECTION ( 'NONE',  ( -0.000000000000000000, 1.000000000000000000, 1.224646799147353207E-16 ) ) ;
#29417=DIRECTION ( 'NONE',  ( 0.000000000000000000, 0.000000000000000000, -1.000000000000000000 ) ) ;
#29458=VERTEX_POINT ( 'NONE', #43503 ) ;
#29461=AXIS2_PLACEMENT_3D ( 'NONE', #63197, #63540, #52627 ) ;
#29543=DIRECTION ( 'NONE',  ( 1.000000000000000000, 0.000000000000000000, 0.000000000000000000 ) ) ;
#29578=ORIENTED_EDGE ( 'NONE', *, *, #64112, .F. ) ;
#29603=CARTESIAN_POINT ( 'NONE',  ( 2.699999999999990408, 0.000000000000000000, -19.99999999999998934 ) ) ;
#29887=CIRCLE ( 'NONE', #68112, 0.3000000000000051514 ) ;
#29940=AXIS2_PLACEMENT_3D ( 'NONE', #8731, #13313, #3441 ) ;
#29959=DIRECTION ( 'NONE',  ( 0.000000000000000000, 0.000000000000000000, 1.000000000000000000 ) ) ;
#29971=VERTEX_POINT ( 'NONE', #25281 ) ;
#30034=( NAMED_UNIT ( * ) PLANE_ANGLE_UNIT ( ) SI_UNIT ( $, .RADIAN. ) );
#30126=CARTESIAN_POINT ( 'NONE',  ( 2.700000000000004619, 0.000000000000000000, 0.000000000000000000 ) ) ;
#30130=DIRECTION ( 'NONE',  ( 1.000000000000000000, 0.000000000000000000, 0.000000000000000000 ) ) ;
#30152=CARTESIAN_POINT ( 'NONE',  ( -2.700000000000004619, 0.000000000000000000, 0.000000000000000000 ) ) ;
#30160=ORIENTED_EDGE ( 'NONE', *, *, #3058, .T. ) ;
#30194=CARTESIAN_POINT ( 'NONE',  ( -20.63749999999999929, 2.449293598294705724E-15, 19.99999999999999289 ) ) ;
#30421=CIRCLE ( 'NONE', #10169, 20.30000000000000071 ) ;
#30628=EDGE_LOOP ( 'NONE', ( #7907, #46578, #58714, #25450 ) ) ;
#30714=VERTEX_POINT ( 'NONE', #32703 ) ;
#30744=DIRECTION ( 'NONE',  ( -1.000000000000000000, 0.000000000000000000, -0.000000000000000000 ) ) ;
#30755=VECTOR ( 'NONE', #17543, 1000.000000000000000 ) ;
#30797=AXIS2_PLACEMENT_3D ( 'NONE', #28562, #3556, #31337 ) ;
#30976=EDGE_LOOP ( 'NONE', ( #7941, #40763 ) ) ;
#31216=ORIENTED_EDGE ( 'NONE', *, *, #51063, .F. ) ;
#31337=DIRECTION ( 'NONE',  ( 0.000000000000000000, 0.000000000000000000, -1.000000000000000000 ) ) ;
#31338=CARTESIAN_POINT ( 'NONE',  ( -2.699999999999990408, 2.449293598294706119E-15, 19.99999999999999645 ) ) ;
#31466=CYLINDRICAL_SURFACE ( 'NONE', #23007, 19.99999999999999289 ) ;
#31480=ORIENTED_EDGE ( 'NONE', *, *, #67117, .T. ) ;
#31540=VERTEX_POINT ( 'NONE', #21803 ) ;
#31790=AXIS2_PLACEMENT_3D ( 'NONE', #33405, #28105, #49199 ) ;
#31797=VERTEX_POINT ( 'NONE', #35147 ) ;
#31843=EDGE_CURVE ( 'NONE', #31540, #53628, #8069, .T. ) ;
#31915=CIRCLE ( 'NONE', #40900, 0.3000000000000051514 ) ;
#31935=EDGE_CURVE ( 'NONE', #61115, #53628, #47006, .T. ) ;
#32051=SHAPE_REPRESENTATION ( 'angular contact ball bearing_68_iso_ISO 15 ABB - 1740 - 38,SI,NC,38_68', ( #66832 ), #621 ) ;
#32142=CARTESIAN_POINT ( 'NONE',  ( -2.700000000000004619, 0.000000000000000000, 0.000000000000000000 ) ) ;
#32161=VECTOR ( 'NONE', #15483, 1000.000000000000000 ) ;
#32258=ORIENTED_EDGE ( 'NONE', *, *, #13977, .F. ) ;
#32660=CIRCLE ( 'NONE', #46166, 0.3000000000000051514 ) ;
#32703=CARTESIAN_POINT ( 'NONE',  ( 3.000000000000006217, 0.000000000000000000, -23.50000000000000000 ) ) ;
#32704=ORIENTED_EDGE ( 'NONE', *, *, #55766, .T. ) ;
#32715=STYLED_ITEM ( 'NONE', ( #5689 ), #17567 ) ;
#32817=AXIS2_PLACEMENT_3D ( 'NONE', #6260, #645, #38624 ) ;
#32830=DIRECTION ( 'NONE',  ( 1.000000000000000000, 0.000000000000000000, 0.000000000000000000 ) ) ;
#32947=VECTOR ( 'NONE', #42954, 1000.000000000000000 ) ;
#33073=DIRECTION ( 'NONE',  ( 1.000000000000000000, 0.000000000000000000, 0.000000000000000000 ) ) ;
#33174=CARTESIAN_POINT ( 'NONE',  ( -0.2727178028659107412, 0.000000000000000000, 0.000000000000000000 ) ) ;
#33244=FACE_OUTER_BOUND ( 'NONE', #4484, .T. ) ;
#33306=ORIENTED_EDGE ( 'NONE', *, *, #6341, .F. ) ;
#33405=CARTESIAN_POINT ( 'NONE',  ( -1.118033988749894458, 0.000000000000000000, 0.000000000000000000 ) ) ;
#33414=VERTEX_POINT ( 'NONE', #35702 ) ;
#33511=VERTEX_POINT ( 'NONE', #59889 ) ;
#33566=DIRECTION ( 'NONE',  ( 0.000000000000000000, 0.000000000000000000, -1.000000000000000000 ) ) ;
#33582=CARTESIAN_POINT ( 'NONE',  ( 0.000000000000000000, 2.755455298081544778E-15, -22.50000000000000000 ) ) ;
#33618=AXIS2_PLACEMENT_3D ( 'NONE', #18277, #61535, #24261 ) ;
#33642=APPLICATION_CONTEXT ( 'automotive_design' ) ;
#33765=FACE_OUTER_BOUND ( 'NONE', #43865, .T. ) ;
#33833=( NAMED_UNIT ( * ) PLANE_ANGLE_UNIT ( ) SI_UNIT ( $, .RADIAN. ) );
#33851=CARTESIAN_POINT ( 'NONE',  ( -20.63749999999999929, 0.000000000000000000, 0.000000000000000000 ) ) ;
#33969=AXIS2_PLACEMENT_3D ( 'NONE', #66841, #2116, #7736 ) ;
#34032=CARTESIAN_POINT ( 'NONE',  ( 0.000000000000000000, 0.000000000000000000, 0.000000000000000000 ) ) ;
#34135=DIRECTION ( 'NONE',  ( 1.000000000000000000, 0.000000000000000000, 0.000000000000000000 ) ) ;
#34143=ORIENTED_EDGE ( 'NONE', *, *, #65424, .T. ) ;
#34179=CARTESIAN_POINT ( 'NONE',  ( -2.999999999999994227, 0.000000000000000000, -20.30000000000000071 ) ) ;
#34180=DIRECTION ( 'NONE',  ( 0.000000000000000000, 0.000000000000000000, -1.000000000000000000 ) ) ;
#34288=ORIENTED_EDGE ( 'NONE', *, *, #36705, .F. ) ;
#34337=CARTESIAN_POINT ( 'NONE',  ( 0.000000000000000000, 0.000000000000000000, 0.000000000000000000 ) ) ;
#34454=DIRECTION ( 'NONE',  ( -1.000000000000000000, -0.000000000000000000, -0.000000000000000000 ) ) ;
#34458=DIRECTION ( 'NONE',  ( 0.000000000000000000, -1.000000000000000000, 0.000000000000000000 ) ) ;
#34528=CARTESIAN_POINT ( 'NONE',  ( -20.63749999999999574, 0.000000000000000000, -23.97499999999999787 ) ) ;
#34569=CARTESIAN_POINT ( 'NONE',  ( -20.63749999999999574, 2.877919977996280320E-15, 23.50000000000000000 ) ) ;
#34661=ORIENTED_EDGE ( 'NONE', *, *, #45920, .T. ) ;
#34673=VECTOR ( 'NONE', #62219, 1000.000000000000000 ) ;
#34781=ORIENTED_EDGE ( 'NONE', *, *, #12227, .F. ) ;
#34822=EDGE_CURVE ( 'NONE', #29971, #33511, #56160, .T. ) ;
#34961=EDGE_CURVE ( 'NONE', #31797, #39615, #19103, .T. ) ;
#34982=AXIS2_PLACEMENT_3D ( 'NONE', #9281, #30744, #2288 ) ;
#35095=ORIENTED_EDGE ( 'NONE', *, *, #63278, .T. ) ;
#35147=CARTESIAN_POINT ( 'NONE',  ( 2.700000000000004619, 0.000000000000000000, -25.00000000000000355 ) ) ;
#35299=ORIENTED_EDGE ( 'NONE', *, *, #38351, .F. ) ;
#35702=CARTESIAN_POINT ( 'NONE',  ( -2.999999999999992450, 0.000000000000000000, -21.50000000000000000 ) ) ;
#35995=AXIS2_PLACEMENT_3D ( 'NONE', #8299, #20565, #8995 ) ;
#36097=PRODUCT_CONTEXT ( 'NONE', #19240, 'mechanical' ) ;
#36138=EDGE_CURVE ( 'NONE', #46466, #19256, #53963, .T. ) ;
#36217=CARTESIAN_POINT ( 'NONE',  ( -20.63749999999999929, 0.000000000000000000, 0.000000000000000000 ) ) ;
#36528=CIRCLE ( 'NONE', #1676, 19.99999999999999645 ) ;
#36705=EDGE_CURVE ( 'NONE', #4257, #19256, #24885, .T. ) ;
#36750=ORIENTED_EDGE ( 'NONE', *, *, #22144, .T. ) ;
#36762=ORIENTED_EDGE ( 'NONE', *, *, #6341, .T. ) ;
#36973=CARTESIAN_POINT ( 'NONE',  ( -20.63749999999999929, 0.000000000000000000, -21.02500000000000213 ) ) ;
#36997=CARTESIAN_POINT ( 'NONE',  ( -2.700000000000004619, 0.000000000000000000, 0.000000000000000000 ) ) ;
#37037=PLANE ( 'NONE',  #53128 ) ;
#37213=CARTESIAN_POINT ( 'NONE',  ( 0.000000000000000000, 0.000000000000000000, 22.50000000000000000 ) ) ;
#37242=ADVANCED_FACE ( 'NONE', ( #33244 ), #27951, .F. ) ;
#37610=CARTESIAN_POINT ( 'NONE',  ( -20.63749999999999574, 3.061616997868383831E-15, 25.00000000000000711 ) ) ;
#37639=EDGE_LOOP ( 'NONE', ( #8081, #8282, #61240, #41098 ) ) ;
#37661=AXIS2_PLACEMENT_3D ( 'NONE', #28962, #32830, #54259 ) ;
#37775=CIRCLE ( 'NONE', #46766, 19.99999999999999645 ) ;
#37822=ADVANCED_FACE ( 'NONE', ( #52771 ), #1323, .T. ) ;
#37898=ORIENTED_EDGE ( 'NONE', *, *, #27397, .T. ) ;
#38076=ADVANCED_FACE ( 'NONE', ( #65078 ), #62025, .T. ) ;
#38093=EDGE_CURVE ( 'NONE', #57773, #42528, #46305, .T. ) ;
#38332=COLOUR_RGB ( '',0.7921568627450980005, 0.8196078431372548767, 0.9333333333333333481 ) ;
#38351=EDGE_CURVE ( 'NONE', #44335, #33511, #8105, .T. ) ;
#38435=ORIENTED_EDGE ( 'NONE', *, *, #62169, .T. ) ;
#38504=EDGE_CURVE ( 'NONE', #33511, #29971, #48529, .T. ) ;
#38593=AXIS2_PLACEMENT_3D ( 'NONE', #45329, #34454, #41698 ) ;
#38610=ADVANCED_FACE ( 'NONE', ( #14649 ), #53065, .T. ) ;
#38624=DIRECTION ( 'NONE',  ( 0.000000000000000000, 0.000000000000000000, 1.000000000000000000 ) ) ;
#38677=CIRCLE ( 'NONE', #31790, 21.50000000000000000 ) ;
#38772=DIRECTION ( 'NONE',  ( 0.000000000000000000, 1.000000000000000000, -1.224646799147353207E-16 ) ) ;
#38941=AXIS2_PLACEMENT_3D ( 'NONE', #49398, #7202, #28662 ) ;
#39113=CARTESIAN_POINT ( 'NONE',  ( -2.699999999999990408, 0.000000000000000000, 0.000000000000000000 ) ) ;
#39189=CIRCLE ( 'NONE', #17843, 19.99999999999998934 ) ;
#39328=CARTESIAN_POINT ( 'NONE',  ( 3.000000000000002665, 0.000000000000000000, -24.69999999999999929 ) ) ;
#39424=CARTESIAN_POINT ( 'NONE',  ( 2.700000000000004619, 0.000000000000000000, 0.000000000000000000 ) ) ;
#39490=EDGE_CURVE ( 'NONE', #57773, #30714, #58447, .T. ) ;
#39615=VERTEX_POINT ( 'NONE', #60886 ) ;
#39630=FACE_OUTER_BOUND ( 'NONE', #5355, .T. ) ;
#39686=AXIS2_PLACEMENT_3D ( 'NONE', #3118, #68180, #47381 ) ;
#39721=CARTESIAN_POINT ( 'NONE',  ( 2.999999999999992450, 0.000000000000000000, -21.02499999999999858 ) ) ;
#39733=CIRCLE ( 'NONE', #30797, 23.50000000000000000 ) ;
#39759=CARTESIAN_POINT ( 'NONE',  ( 2.700000000000004619, 0.000000000000000000, 0.000000000000000000 ) ) ;
#39782=EDGE_CURVE ( 'NONE', #27706, #61321, #23614, .T. ) ;
#39856=EDGE_CURVE ( 'NONE', #29971, #31797, #60458, .T. ) ;
#39876=AXIS2_PLACEMENT_3D ( 'NONE', #36217, #58016, #52394 ) ;
#39968=DIRECTION ( 'NONE',  ( 1.000000000000000000, 0.000000000000000000, 0.000000000000000000 ) ) ;
#40250=ORIENTED_EDGE ( 'NONE', *, *, #51153, .F. ) ;
#40286=ADVANCED_FACE ( 'NONE', ( #8307 ), #6069, .T. ) ;
#40469=ORIENTED_EDGE ( 'NONE', *, *, #39782, .T. ) ;
#40473=CARTESIAN_POINT ( 'NONE',  ( -3.000000000000006217, 0.000000000000000000, -23.97499999999999787 ) ) ;
#40560=DIRECTION ( 'NONE',  ( 0.000000000000000000, 0.000000000000000000, -1.000000000000000000 ) ) ;
#40763=ORIENTED_EDGE ( 'NONE', *, *, #27397, .F. ) ;
#40811=EDGE_CURVE ( 'NONE', #53628, #61115, #38677, .T. ) ;
#40900=AXIS2_PLACEMENT_3D ( 'NONE', #57907, #53648, #25907 ) ;
#40996=TOROIDAL_SURFACE ( 'NONE', #67968, 20.30000000000000071, 0.3000000000000062061 ) ;
#41098=ORIENTED_EDGE ( 'NONE', *, *, #40811, .T. ) ;
#41130=ADVANCED_FACE ( 'NONE', ( #39630 ), #28479, .T. ) ;
#41144=ORIENTED_EDGE ( 'NONE', *, *, #28417, .F. ) ;
#41248=AXIS2_PLACEMENT_3D ( 'NONE', #18946, #56574, #8749 ) ;
#41372=ADVANCED_FACE ( 'NONE', ( #49731 ), #53621, .T. ) ;
#41435=LINE ( 'NONE', #30194, #26234 ) ;
#41641=ORIENTED_EDGE ( 'NONE', *, *, #55766, .F. ) ;
#41679=DIRECTION ( 'NONE',  ( 0.000000000000000000, 0.000000000000000000, -1.000000000000000000 ) ) ;
#41698=DIRECTION ( 'NONE',  ( 0.000000000000000000, 0.000000000000000000, 1.000000000000000000 ) ) ;
#41756=EDGE_CURVE ( 'NONE', #30714, #60665, #39733, .T. ) ;
#41822=CLOSED_SHELL ( 'NONE', ( #57806, #60125, #38610, #51690, #61403, #43338, #38076, #43924, #23960, #69470, #41372, #18451, #2799, #42960, #25517, #14748, #40286, #43419, #25190, #18903, #37822, #52898, #37242, #57648, #64457, #41130, #4152, #28025 ) ) ;
#42027=EDGE_CURVE ( 'NONE', #29458, #61321, #18384, .T. ) ;
#42211=LINE ( 'NONE', #37610, #32161 ) ;
#42303=AXIS2_PLACEMENT_3D ( 'NONE', #56310, #50689, #34180 ) ;
#42497=DIRECTION ( 'NONE',  ( 0.000000000000000000, 0.000000000000000000, -1.000000000000000000 ) ) ;
#42528=VERTEX_POINT ( 'NONE', #14664 ) ;
#42531=AXIS2_PLACEMENT_3D ( 'NONE', #54449, #6278, #61494 ) ;
#42578=ORIENTED_EDGE ( 'NONE', *, *, #3058, .F. ) ;
#42663=VECTOR ( 'NONE', #17532, 1000.000000000000000 ) ;
#42917=ORIENTED_EDGE ( 'NONE', *, *, #63278, .F. ) ;
#42954=DIRECTION ( 'NONE',  ( 1.000000000000000000, 0.000000000000000000, 0.000000000000000000 ) ) ;
#42960=ADVANCED_FACE ( 'NONE', ( #48456 ), #290, .T. ) ;
#43325=AXIS2_PLACEMENT_3D ( 'NONE', #4680, #26146, #24770 ) ;
#43338=ADVANCED_FACE ( 'NONE', ( #8641 ), #27450, .T. ) ;
#43371=CARTESIAN_POINT ( 'NONE',  ( 3.000000000000002665, 3.043247295881173007E-15, 24.69999999999999929 ) ) ;
#43419=ADVANCED_FACE ( 'NONE', ( #46952 ), #31466, .F. ) ;
#43503=CARTESIAN_POINT ( 'NONE',  ( -0.2727178028659107967, 0.000000000000000000, 23.97499999999999787 ) ) ;
#43841=FACE_OUTER_BOUND ( 'NONE', #51328, .T. ) ;
#43865=EDGE_LOOP ( 'NONE', ( #53387, #5423, #66121, #42917 ) ) ;
#43924=ADVANCED_FACE ( 'NONE', ( #19854 ), #67363, .F. ) ;
#44081=DIRECTION ( 'NONE',  ( 1.000000000000000000, 0.000000000000000000, 0.000000000000000000 ) ) ;
#44141=CIRCLE ( 'NONE', #7109, 21.02500000000000213 ) ;
#44335=VERTEX_POINT ( 'NONE', #62611 ) ;
#44558=DIRECTION ( 'NONE',  ( 0.000000000000000000, 0.000000000000000000, 1.000000000000000000 ) ) ;
#44563=DIRECTION ( 'NONE',  ( 0.000000000000000000, 0.000000000000000000, -1.000000000000000000 ) ) ;
#44682=DIRECTION ( 'NONE',  ( 0.000000000000000000, 0.000000000000000000, 1.000000000000000000 ) ) ;
#44726=DIRECTION ( 'NONE',  ( 0.000000000000000000, 0.000000000000000000, -1.000000000000000000 ) ) ;
#44872=DIRECTION ( 'NONE',  ( 0.000000000000000000, 0.000000000000000000, -1.000000000000000000 ) ) ;
#44989=CARTESIAN_POINT ( 'NONE',  ( -2.999999999999992450, 0.000000000000000000, 0.000000000000000000 ) ) ;
#45104=DIRECTION ( 'NONE',  ( 0.000000000000000000, 0.000000000000000000, -1.000000000000000000 ) ) ;
#45151=UNCERTAINTY_MEASURE_WITH_UNIT (LENGTH_MEASURE( 1.000000000000000082E-05 ), #57453, 'distance_accuracy_value', 'NONE');
#45223=CIRCLE ( 'NONE', #54179, 23.97499999999999787 ) ;
#45309=CARTESIAN_POINT ( 'NONE',  ( 2.999999999999996003, 2.486033002269127373E-15, 20.30000000000000071 ) ) ;
#45329=CARTESIAN_POINT ( 'NONE',  ( 0.000000000000000000, 0.000000000000000000, 0.000000000000000000 ) ) ;
#45379=DIRECTION ( 'NONE',  ( 0.000000000000000000, -1.224646799147351975E-16, 1.000000000000000000 ) ) ;
#45411=AXIS2_PLACEMENT_3D ( 'NONE', #10939, #34458, #49908 ) ;
#45518=EDGE_CURVE ( 'NONE', #54364, #29971, #29887, .T. ) ;
#45582=ORIENTED_EDGE ( 'NONE', *, *, #5645, .T. ) ;
#45658=CIRCLE ( 'NONE', #46808, 0.3000000000000051514 ) ;
#45848=ADVANCED_BREP_SHAPE_REPRESENTATION ( '', ( #17567, #66832 ), #621 ) ;
#45920=EDGE_CURVE ( 'NONE', #19652, #42528, #1879, .T. ) ;
#46063=AXIS2_PLACEMENT_3D ( 'NONE', #36997, #6372, #16224 ) ;
#46143=ORIENTED_EDGE ( 'NONE', *, *, #5645, .F. ) ;
#46166=AXIS2_PLACEMENT_3D ( 'NONE', #64493, #64843, #5737 ) ;
#46248=DIRECTION ( 'NONE',  ( -1.000000000000000000, -0.000000000000000000, -0.000000000000000000 ) ) ;
#46253=DIRECTION ( 'NONE',  ( 1.000000000000000000, 0.000000000000000000, 0.000000000000000000 ) ) ;
#46257=CARTESIAN_POINT ( 'NONE',  ( -2.999999999999992450, 0.000000000000000000, 0.000000000000000000 ) ) ;
#46287=EDGE_LOOP ( 'NONE', ( #52292, #38435, #63147, #69258 ) ) ;
#46305=CIRCLE ( 'NONE', #33969, 23.50000000000000000 ) ;
#46466=VERTEX_POINT ( 'NONE', #34179 ) ;
#46563=PLANE ( 'NONE',  #34982 ) ;
#46578=ORIENTED_EDGE ( 'NONE', *, *, #9301, .T. ) ;
#46766=AXIS2_PLACEMENT_3D ( 'NONE', #39113, #55267, #44726 ) ;
#46808=AXIS2_PLACEMENT_3D ( 'NONE', #8764, #51324, #14023 ) ;
#46952=FACE_OUTER_BOUND ( 'NONE', #14189, .T. ) ;
#47006=CIRCLE ( 'NONE', #16665, 21.50000000000000000 ) ;
#47381=DIRECTION ( 'NONE',  ( 0.000000000000000000, 0.000000000000000000, -1.000000000000000000 ) ) ;
#47753=CARTESIAN_POINT ( 'NONE',  ( 0.2727178028659107412, 2.726369936601795653E-15, -21.02500000000000213 ) ) ;
#47766=CARTESIAN_POINT ( 'NONE',  ( -1.118033988749894458, 0.000000000000000000, 0.000000000000000000 ) ) ;
#47769=DIRECTION ( 'NONE',  ( 0.000000000000000000, 1.224646799147344826E-16, 1.000000000000000000 ) ) ;
#47897=CIRCLE ( 'NONE', #54624, 21.50000000000000000 ) ;
#47990=ORIENTED_EDGE ( 'NONE', *, *, #31843, .T. ) ;
#48179=ORIENTED_EDGE ( 'NONE', *, *, #34822, .F. ) ;
#48241=FILL_AREA_STYLE_COLOUR ( '', #38332 ) ;
#48456=FACE_OUTER_BOUND ( 'NONE', #2981, .T. ) ;
#48476=CARTESIAN_POINT ( 'NONE',  ( -20.63749999999999574, 0.000000000000000000, -25.00000000000000711 ) ) ;
#48529=CIRCLE ( 'NONE', #18246, 25.00000000000000711 ) ;
#48562=ORIENTED_EDGE ( 'NONE', *, *, #23576, .T. ) ;
#48639=VECTOR ( 'NONE', #65478, 1000.000000000000000 ) ;
#48643=DIRECTION ( 'NONE',  ( 0.000000000000000000, 0.000000000000000000, -1.000000000000000000 ) ) ;
#48770=EDGE_LOOP ( 'NONE', ( #66582, #24277 ) ) ;
#48934=( LENGTH_UNIT ( ) NAMED_UNIT ( * ) SI_UNIT ( .MILLI., .METRE. ) );
#49076=CARTESIAN_POINT ( 'NONE',  ( 2.999999999999996003, 0.000000000000000000, -20.30000000000000071 ) ) ;
#49185=DIRECTION ( 'NONE',  ( -1.000000000000000000, 0.000000000000000000, -0.000000000000000000 ) ) ;
#49199=DIRECTION ( 'NONE',  ( 0.000000000000000000, 0.000000000000000000, -1.000000000000000000 ) ) ;
#49263=DIRECTION ( 'NONE',  ( 0.000000000000000000, 0.000000000000000000, -1.000000000000000000 ) ) ;
#49271=LINE ( 'NONE', #1105, #48639 ) ;
#49392=DIRECTION ( 'NONE',  ( 0.000000000000000000, 0.000000000000000000, -1.000000000000000000 ) ) ;
#49398=CARTESIAN_POINT ( 'NONE',  ( -3.000000000000002665, 0.000000000000000000, 0.000000000000000000 ) ) ;
#49556=EDGE_LOOP ( 'NONE', ( #51286, #45582, #56430, #20081 ) ) ;
#49632=CYLINDRICAL_SURFACE ( 'NONE', #4739, 23.50000000000000000 ) ;
#49641=SURFACE_STYLE_USAGE ( .BOTH. , #1469 ) ;
#49656=AXIS2_PLACEMENT_3D ( 'NONE', #27347, #6245, #47769 ) ;
#49731=FACE_OUTER_BOUND ( 'NONE', #53930, .T. ) ;
#49759=CARTESIAN_POINT ( 'NONE',  ( 2.999999999999992450, 2.574819895207310198E-15, 21.02499999999999858 ) ) ;
#49790=VERTEX_POINT ( 'NONE', #24957 ) ;
#49908=DIRECTION ( 'NONE',  ( 0.000000000000000000, 0.000000000000000000, -1.000000000000000000 ) ) ;
#49938=EDGE_CURVE ( 'NONE', #29458, #53628, #54766, .T. ) ;
#50316=DIRECTION ( 'NONE',  ( 0.000000000000000000, 0.000000000000000000, -1.000000000000000000 ) ) ;
#50530=CARTESIAN_POINT ( 'NONE',  ( 0.000000000000000000, 0.000000000000000000, 0.000000000000000000 ) ) ;
#50689=DIRECTION ( 'NONE',  ( 1.000000000000000000, 0.000000000000000000, 0.000000000000000000 ) ) ;
#51018=VERTEX_POINT ( 'NONE', #43371 ) ;
#51063=EDGE_CURVE ( 'NONE', #25778, #46466, #32660, .T. ) ;
#51081=AXIS2_PLACEMENT_3D ( 'NONE', #34337, #46248, #67727 ) ;
#51153=EDGE_CURVE ( 'NONE', #66051, #17861, #57421, .T. ) ;
#51162=DIRECTION ( 'NONE',  ( 1.000000000000000000, 0.000000000000000000, 0.000000000000000000 ) ) ;
#51171=ORIENTED_EDGE ( 'NONE', *, *, #21650, .T. ) ;
#51286=ORIENTED_EDGE ( 'NONE', *, *, #8768, .T. ) ;
#51317=ORIENTED_EDGE ( 'NONE', *, *, #28417, .T. ) ;
#51324=DIRECTION ( 'NONE',  ( 0.000000000000000000, -1.000000000000000000, 0.000000000000000000 ) ) ;
#51328=EDGE_LOOP ( 'NONE', ( #23340, #47990, #16904, #41641 ) ) ;
#51646=DIRECTION ( 'NONE',  ( 1.000000000000000000, 0.000000000000000000, 0.000000000000000000 ) ) ;
#51690=ADVANCED_FACE ( 'NONE', ( #16734 ), #12172, .F. ) ;
#51793=DIRECTION ( 'NONE',  ( 1.000000000000000000, 0.000000000000000000, 0.000000000000000000 ) ) ;
#52019=CARTESIAN_POINT ( 'NONE',  ( -20.63749999999999929, 2.632990618166809235E-15, 21.50000000000000000 ) ) ;
#52108=DIRECTION ( 'NONE',  ( 1.000000000000000000, 0.000000000000000000, 0.000000000000000000 ) ) ;
#52177=DIRECTION ( 'NONE',  ( -1.000000000000000000, -0.000000000000000000, -0.000000000000000000 ) ) ;
#52292=ORIENTED_EDGE ( 'NONE', *, *, #27150, .F. ) ;
#52394=DIRECTION ( 'NONE',  ( 0.000000000000000000, 0.000000000000000000, -1.000000000000000000 ) ) ;
#52504=CARTESIAN_POINT ( 'NONE',  ( 2.999999999999993339, 20.30000000000000071, 0.000000000000000000 ) ) ;
#52524=ORIENTED_EDGE ( 'NONE', *, *, #14434, .F. ) ;
#52559=VERTEX_POINT ( 'NONE', #45309 ) ;
#52627=DIRECTION ( 'NONE',  ( 0.000000000000000000, 0.000000000000000000, -1.000000000000000000 ) ) ;
#52771=FACE_OUTER_BOUND ( 'NONE', #37639, .T. ) ;
#52848=DIRECTION ( 'NONE',  ( 1.000000000000000000, 0.000000000000000000, 0.000000000000000000 ) ) ;
#52898=ADVANCED_FACE ( 'NONE', ( #54909 ), #49632, .F. ) ;
#53039=ORIENTED_EDGE ( 'NONE', *, *, #3880, .T. ) ;
#53062=ORIENTED_EDGE ( 'NONE', *, *, #8768, .F. ) ;
#53065=TOROIDAL_SURFACE ( 'NONE', #1417, 24.69999999999999929, 0.3000000000000035971 ) ;
#53128=AXIS2_PLACEMENT_3D ( 'NONE', #16263, #52848, #4670 ) ;
#53256=ORIENTED_EDGE ( 'NONE', *, *, #8961, .T. ) ;
#53353=DIRECTION ( 'NONE',  ( 1.000000000000000000, 0.000000000000000000, 0.000000000000000000 ) ) ;
#53376=TOROIDAL_SURFACE ( 'NONE', #37661, 24.69999999999999929, 0.3000000000000035971 ) ;
#53381=DIRECTION ( 'NONE',  ( 0.000000000000000000, -1.000000000000000000, 0.000000000000000000 ) ) ;
#53387=ORIENTED_EDGE ( 'NONE', *, *, #9009, .F. ) ;
#53532=PRODUCT_DEFINITION_CONTEXT ( 'detailed design', #33642, 'design' ) ;
#53621=CYLINDRICAL_SURFACE ( 'NONE', #22853, 21.02500000000000213 ) ;
#53628=VERTEX_POINT ( 'NONE', #16344 ) ;
#53648=DIRECTION ( 'NONE',  ( 0.000000000000000000, 1.000000000000000000, -1.224646799147353207E-16 ) ) ;
#53667=AXIS2_PLACEMENT_3D ( 'NONE', #39759, #29543, #50316 ) ;
#53928=DIRECTION ( 'NONE',  ( 1.000000000000000000, 0.000000000000000000, 0.000000000000000000 ) ) ;
#53930=EDGE_LOOP ( 'NONE', ( #60593, #9888, #8902, #55653 ) ) ;
#53963=CIRCLE ( 'NONE', #5676, 20.30000000000000071 ) ;
#53989=ORIENTED_EDGE ( 'NONE', *, *, #9009, .T. ) ;
#54179=AXIS2_PLACEMENT_3D ( 'NONE', #10835, #6953, #6250 ) ;
#54237=ORIENTED_EDGE ( 'NONE', *, *, #8961, .F. ) ;
#54259=DIRECTION ( 'NONE',  ( 0.000000000000000000, 0.000000000000000000, -1.000000000000000000 ) ) ;
#54351=ORIENTED_EDGE ( 'NONE', *, *, #51153, .T. ) ;
#54364=VERTEX_POINT ( 'NONE', #11493 ) ;
#54383=AXIS2_PLACEMENT_3D ( 'NONE', #66501, #34135, #44682 ) ;
#54411=FACE_OUTER_BOUND ( 'NONE', #18974, .T. ) ;
#54449=CARTESIAN_POINT ( 'NONE',  ( 2.700000000000004619, 3.024877593893962577E-15, 24.69999999999999929 ) ) ;
#54462=FACE_BOUND ( 'NONE', #25930, .T. ) ;
#54488=ORIENTED_EDGE ( 'NONE', *, *, #23576, .F. ) ;
#54500=DIRECTION ( 'NONE',  ( 0.000000000000000000, 0.000000000000000000, -1.000000000000000000 ) ) ;
#54624=AXIS2_PLACEMENT_3D ( 'NONE', #44989, #3137, #61852 ) ;
#54715=DIRECTION ( 'NONE',  ( 1.000000000000000000, 0.000000000000000000, 0.000000000000000000 ) ) ;
#54766=CIRCLE ( 'NONE', #64922, 1.500000000000001332 ) ;
#54909=FACE_OUTER_BOUND ( 'NONE', #17319, .T. ) ;
#54920=( NAMED_UNIT ( * ) SI_UNIT ( $, .STERADIAN. ) SOLID_ANGLE_UNIT ( ) );
#54952=DIRECTION ( 'NONE',  ( 1.000000000000000000, 0.000000000000000000, 0.000000000000000000 ) ) ;
#55008=DIRECTION ( 'NONE',  ( -0.000000000000000000, 1.000000000000000000, 1.224646799147353207E-16 ) ) ;
#55030=VERTEX_POINT ( 'NONE', #29603 ) ;
#55267=DIRECTION ( 'NONE',  ( 1.000000000000000000, 0.000000000000000000, 0.000000000000000000 ) ) ;
#55275=SURFACE_STYLE_FILL_AREA ( #10277 ) ;
#55292=FACE_OUTER_BOUND ( 'NONE', #9905, .T. ) ;
#55451=DIRECTION ( 'NONE',  ( 1.000000000000000000, 0.000000000000000000, 0.000000000000000000 ) ) ;
#55475=ORIENTED_EDGE ( 'NONE', *, *, #15387, .F. ) ;
#55642=CYLINDRICAL_SURFACE ( 'NONE', #660, 21.50000000000000000 ) ;
#55653=ORIENTED_EDGE ( 'NONE', *, *, #65595, .F. ) ;
#55766=EDGE_CURVE ( 'NONE', #33414, #61115, #16286, .T. ) ;
#55822=AXIS2_PLACEMENT_3D ( 'NONE', #24286, #29206, #45379 ) ;
#56006=DIRECTION ( 'NONE',  ( 0.000000000000000000, 0.000000000000000000, -1.000000000000000000 ) ) ;
#56139=CARTESIAN_POINT ( 'NONE',  ( 2.699999999999990408, 0.000000000000000000, 0.000000000000000000 ) ) ;
#56152=DIRECTION ( 'NONE',  ( 1.000000000000000000, 0.000000000000000000, 0.000000000000000000 ) ) ;
#56160=CIRCLE ( 'NONE', #46063, 25.00000000000000711 ) ;
#56271=AXIS2_PLACEMENT_3D ( 'NONE', #9922, #51793, #68987 ) ;
#56310=CARTESIAN_POINT ( 'NONE',  ( 2.999999999999995559, 0.000000000000000000, 0.000000000000000000 ) ) ;
#56430=ORIENTED_EDGE ( 'NONE', *, *, #23031, .F. ) ;
#56574=DIRECTION ( 'NONE',  ( 1.000000000000000000, 0.000000000000000000, 0.000000000000000000 ) ) ;
#56771=DIRECTION ( 'NONE',  ( 0.000000000000000000, 0.000000000000000000, 1.000000000000000000 ) ) ;
#56848=PRODUCT_DEFINITION ( 'UNKNOWN', '', #57964, #53532 ) ;
#57421=CIRCLE ( 'NONE', #27077, 21.02499999999999858 ) ;
#57453=( LENGTH_UNIT ( ) NAMED_UNIT ( * ) SI_UNIT ( .MILLI., .METRE. ) );
#57567=DIRECTION ( 'NONE',  ( 0.000000000000000000, 0.000000000000000000, -1.000000000000000000 ) ) ;
#57648=ADVANCED_FACE ( 'NONE', ( #10671 ), #28700, .T. ) ;
#57773=VERTEX_POINT ( 'NONE', #68726 ) ;
#57806=ADVANCED_FACE ( 'NONE', ( #21574 ), #53376, .T. ) ;
#57885=CARTESIAN_POINT ( 'NONE',  ( -20.63749999999999574, 0.000000000000000000, 0.000000000000000000 ) ) ;
#57890=SHAPE_DEFINITION_REPRESENTATION ( #4593, #32051 ) ;
#57907=CARTESIAN_POINT ( 'NONE',  ( 2.699999999999990408, 2.486033002269127373E-15, 20.30000000000000071 ) ) ;
#57964=PRODUCT_DEFINITION_FORMATION_WITH_SPECIFIED_SOURCE ( 'ANY', '', #26510, .NOT_KNOWN. ) ;
#58016=DIRECTION ( 'NONE',  ( 1.000000000000000000, 0.000000000000000000, 0.000000000000000000 ) ) ;
#58165=EDGE_LOOP ( 'NONE', ( #33306, #34143, #37898, #7160 ) ) ;
#58252=EDGE_LOOP ( 'NONE', ( #46143, #13239, #6152, #17193 ) ) ;
#58447=LINE ( 'NONE', #27133, #32947 ) ;
#58676=DIRECTION ( 'NONE',  ( 0.000000000000000000, 0.000000000000000000, -1.000000000000000000 ) ) ;
#58701=ORIENTED_EDGE ( 'NONE', *, *, #12227, .T. ) ;
#58704=CIRCLE ( 'NONE', #3692, 1.500000000000001332 ) ;
#58714=ORIENTED_EDGE ( 'NONE', *, *, #31935, .T. ) ;
#58804=ORIENTED_EDGE ( 'NONE', *, *, #34822, .T. ) ;
#58822=FACE_BOUND ( 'NONE', #30976, .T. ) ;
#58848=EDGE_CURVE ( 'NONE', #4257, #25778, #36528, .T. ) ;
#59093=CARTESIAN_POINT ( 'NONE',  ( -2.699999999999990408, 0.000000000000000000, -19.99999999999999645 ) ) ;
#59635=CARTESIAN_POINT ( 'NONE',  ( -20.63749999999999574, 0.000000000000000000, 0.000000000000000000 ) ) ;
#59658=( GEOMETRIC_REPRESENTATION_CONTEXT ( 3 ) GLOBAL_UNCERTAINTY_ASSIGNED_CONTEXT ( ( #25456 ) ) GLOBAL_UNIT_ASSIGNED_CONTEXT ( ( #48934, #33833, #54920 ) ) REPRESENTATION_CONTEXT ( 'NONE', 'WORKASPACE' ) );
#59889=CARTESIAN_POINT ( 'NONE',  ( -2.700000000000004619, 3.061616997868383831E-15, 25.00000000000000711 ) ) ;
#60056=AXIS2_PLACEMENT_3D ( 'NONE', #69198, #53353, #65319 ) ;
#60125=ADVANCED_FACE ( 'NONE', ( #24845 ), #68110, .T. ) ;
#60157=TOROIDAL_SURFACE ( 'NONE', #43325, 20.30000000000000071, 0.3000000000000062061 ) ;
#60245=DIRECTION ( 'NONE',  ( -1.000000000000000000, -0.000000000000000000, -0.000000000000000000 ) ) ;
#60458=LINE ( 'NONE', #48476, #30755 ) ;
#60565=DIRECTION ( 'NONE',  ( 0.000000000000000000, 1.224646799147357891E-16, 1.000000000000000000 ) ) ;
#60593=ORIENTED_EDGE ( 'NONE', *, *, #3880, .F. ) ;
#60665=VERTEX_POINT ( 'NONE', #15589 ) ;
#60786=DIRECTION ( 'NONE',  ( 1.000000000000000000, 0.000000000000000000, 0.000000000000000000 ) ) ;
#60812=VERTEX_POINT ( 'NONE', #47753 ) ;
#60875=DIRECTION ( 'NONE',  ( 1.000000000000000000, 0.000000000000000000, 0.000000000000000000 ) ) ;
#60886=CARTESIAN_POINT ( 'NONE',  ( 2.700000000000004619, 3.061616997868383437E-15, 25.00000000000000355 ) ) ;
#61034=ORIENTED_EDGE ( 'NONE', *, *, #58848, .F. ) ;
#61115=VERTEX_POINT ( 'NONE', #15676 ) ;
#61121=AXIS2_PLACEMENT_3D ( 'NONE', #56139, #8658, #61421 ) ;
#61240=ORIENTED_EDGE ( 'NONE', *, *, #49938, .T. ) ;
#61281=DIRECTION ( 'NONE',  ( 1.000000000000000000, 0.000000000000000000, 0.000000000000000000 ) ) ;
#61298=EDGE_CURVE ( 'NONE', #54364, #44335, #21001, .T. ) ;
#61321=VERTEX_POINT ( 'NONE', #1943 ) ;
#61403=ADVANCED_FACE ( 'NONE', ( #8602 ), #4007, .F. ) ;
#61421=DIRECTION ( 'NONE',  ( 0.000000000000000000, 0.000000000000000000, -1.000000000000000000 ) ) ;
#61494=DIRECTION ( 'NONE',  ( 0.000000000000000000, 1.224646799147344826E-16, 1.000000000000000000 ) ) ;
#61535=DIRECTION ( 'NONE',  ( 1.000000000000000000, 0.000000000000000000, 0.000000000000000000 ) ) ;
#61611=CARTESIAN_POINT ( 'NONE',  ( -2.699999999999990408, 2.486033002269127373E-15, 20.30000000000000071 ) ) ;
#61744=DIRECTION ( 'NONE',  ( 1.000000000000000000, 0.000000000000000000, 0.000000000000000000 ) ) ;
#61852=DIRECTION ( 'NONE',  ( 0.000000000000000000, 0.000000000000000000, -1.000000000000000000 ) ) ;
#62025=TOROIDAL_SURFACE ( 'NONE', #12629, 20.30000000000000071, 0.3000000000000062061 ) ;
#62122=ORIENTED_EDGE ( 'NONE', *, *, #27150, .T. ) ;
#62169=EDGE_CURVE ( 'NONE', #49790, #29458, #20189, .T. ) ;
#62219=DIRECTION ( 'NONE',  ( 1.000000000000000000, 0.000000000000000000, 0.000000000000000000 ) ) ;
#62611=CARTESIAN_POINT ( 'NONE',  ( -3.000000000000002665, 3.043247295881173007E-15, 24.69999999999999929 ) ) ;
#63102=CARTESIAN_POINT ( 'NONE',  ( -20.63749999999999574, 2.936090700955778569E-15, 23.97499999999999787 ) ) ;
#63132=DIRECTION ( 'NONE',  ( 1.000000000000000000, 0.000000000000000000, 0.000000000000000000 ) ) ;
#63147=ORIENTED_EDGE ( 'NONE', *, *, #373, .F. ) ;
#63156=CIRCLE ( 'NONE', #32817, 21.02500000000000213 ) ;
#63197=CARTESIAN_POINT ( 'NONE',  ( 2.999999999999995559, 0.000000000000000000, 0.000000000000000000 ) ) ;
#63244=CIRCLE ( 'NONE', #23978, 21.50000000000000000 ) ;
#63278=EDGE_CURVE ( 'NONE', #39615, #31797, #2038, .T. ) ;
#63291=CIRCLE ( 'NONE', #39686, 21.02499999999999858 ) ;
#63339=ORIENTED_EDGE ( 'NONE', *, *, #38504, .F. ) ;
#63540=DIRECTION ( 'NONE',  ( 1.000000000000000000, 0.000000000000000000, 0.000000000000000000 ) ) ;
#64107=SHAPE_REPRESENTATION_RELATIONSHIP ( 'NONE' , 'NONE' ,  #32051, #45848 ) ;
#64112=EDGE_CURVE ( 'NONE', #39615, #51018, #969, .T. ) ;
#64153=EDGE_CURVE ( 'NONE', #6514, #55030, #39189, .T. ) ;
#64310=DIRECTION ( 'NONE',  ( 1.000000000000000000, 0.000000000000000000, 0.000000000000000000 ) ) ;
#64457=ADVANCED_FACE ( 'NONE', ( #33765 ), #2447, .T. ) ;
#64493=CARTESIAN_POINT ( 'NONE',  ( -2.699999999999990408, 0.000000000000000000, -20.30000000000000071 ) ) ;
#64535=CARTESIAN_POINT ( 'NONE',  ( -20.63749999999999929, 0.000000000000000000, 0.000000000000000000 ) ) ;
#64545=ORIENTED_EDGE ( 'NONE', *, *, #38093, .F. ) ;
#64613=DIRECTION ( 'NONE',  ( 0.000000000000000000, 0.000000000000000000, -1.000000000000000000 ) ) ;
#64843=DIRECTION ( 'NONE',  ( 0.000000000000000000, -1.000000000000000000, 0.000000000000000000 ) ) ;
#64861=ORIENTED_EDGE ( 'NONE', *, *, #31843, .F. ) ;
#64922=AXIS2_PLACEMENT_3D ( 'NONE', #37213, #53381, #26670 ) ;
#64973=CYLINDRICAL_SURFACE ( 'NONE', #60056, 21.50000000000000000 ) ;
#65078=FACE_OUTER_BOUND ( 'NONE', #1055, .T. ) ;
#65146=AXIS2_PLACEMENT_3D ( 'NONE', #39424, #60875, #7431 ) ;
#65307=AXIS2_PLACEMENT_3D ( 'NONE', #59635, #54715, #44872 ) ;
#65319=DIRECTION ( 'NONE',  ( 0.000000000000000000, 0.000000000000000000, -1.000000000000000000 ) ) ;
#65424=EDGE_CURVE ( 'NONE', #42528, #60665, #2890, .T. ) ;
#65478=DIRECTION ( 'NONE',  ( 1.000000000000000000, 0.000000000000000000, 0.000000000000000000 ) ) ;
#65595=EDGE_CURVE ( 'NONE', #60812, #17861, #22432, .T. ) ;
#65906=CARTESIAN_POINT ( 'NONE',  ( 2.999999999999992450, 0.000000000000000000, 0.000000000000000000 ) ) ;
#66051=VERTEX_POINT ( 'NONE', #49759 ) ;
#66121=ORIENTED_EDGE ( 'NONE', *, *, #39856, .T. ) ;
#66407=DIRECTION ( 'NONE',  ( 0.000000000000000000, 0.000000000000000000, 1.000000000000000000 ) ) ;
#66441=ORIENTED_EDGE ( 'NONE', *, *, #34961, .F. ) ;
#66501=CARTESIAN_POINT ( 'NONE',  ( 1.118033988749894458, 0.000000000000000000, 0.000000000000000000 ) ) ;
#66582=ORIENTED_EDGE ( 'NONE', *, *, #61298, .F. ) ;
#66832=AXIS2_PLACEMENT_3D ( 'NONE', #50530, #44558, #8319 ) ;
#66837=CIRCLE ( 'NONE', #54383, 23.50000000000000000 ) ;
#66841=CARTESIAN_POINT ( 'NONE',  ( 1.118033988749894458, 0.000000000000000000, 0.000000000000000000 ) ) ;
#66903=DIRECTION ( 'NONE',  ( 1.000000000000000000, 0.000000000000000000, 0.000000000000000000 ) ) ;
#66976=DIRECTION ( 'NONE',  ( 0.000000000000000000, 0.000000000000000000, -1.000000000000000000 ) ) ;
#67117=EDGE_CURVE ( 'NONE', #60812, #19652, #63156, .T. ) ;
#67247=VERTEX_POINT ( 'NONE', #39328 ) ;
#67277=ORIENTED_EDGE ( 'NONE', *, *, #58848, .T. ) ;
#67320=DIRECTION ( 'NONE',  ( 1.000000000000000000, 0.000000000000000000, 0.000000000000000000 ) ) ;
#67323=EDGE_LOOP ( 'NONE', ( #36750, #54351 ) ) ;
#67363=CYLINDRICAL_SURFACE ( 'NONE', #16318, 19.99999999999999289 ) ;
#67535=EDGE_CURVE ( 'NONE', #19652, #66051, #49271, .T. ) ;
#67546=ORIENTED_EDGE ( 'NONE', *, *, #13977, .T. ) ;
#67727=DIRECTION ( 'NONE',  ( 0.000000000000000000, 0.000000000000000000, 1.000000000000000000 ) ) ;
#67968=AXIS2_PLACEMENT_3D ( 'NONE', #2692, #56152, #44563 ) ;
#68051=DIRECTION ( 'NONE',  ( 0.000000000000000000, 0.000000000000000000, -1.000000000000000000 ) ) ;
#68069=AXIS2_PLACEMENT_3D ( 'NONE', #57885, #30130, #19561 ) ;
#68110=CYLINDRICAL_SURFACE ( 'NONE', #68069, 25.00000000000000711 ) ;
#68112=AXIS2_PLACEMENT_3D ( 'NONE', #23260, #2492, #49263 ) ;
#68180=DIRECTION ( 'NONE',  ( 1.000000000000000000, 0.000000000000000000, 0.000000000000000000 ) ) ;
#68269=ORIENTED_EDGE ( 'NONE', *, *, #22230, .F. ) ;
#68279=EDGE_LOOP ( 'NONE', ( #53062, #1945 ) ) ;
#68726=CARTESIAN_POINT ( 'NONE',  ( 1.118033988749894458, 2.877919977996280320E-15, -23.50000000000000000 ) ) ;
#68736=CARTESIAN_POINT ( 'NONE',  ( -20.63749999999999929, 0.000000000000000000, 0.000000000000000000 ) ) ;
#68953=CARTESIAN_POINT ( 'NONE',  ( 0.000000000000000000, 0.000000000000000000, 0.000000000000000000 ) ) ;
#68987=DIRECTION ( 'NONE',  ( 0.000000000000000000, 0.000000000000000000, -1.000000000000000000 ) ) ;
#69063=DIRECTION ( 'NONE',  ( 0.000000000000000000, 0.000000000000000000, -1.000000000000000000 ) ) ;
#69191=CIRCLE ( 'NONE', #11898, 24.69999999999999929 ) ;
#69198=CARTESIAN_POINT ( 'NONE',  ( -20.63749999999999929, 0.000000000000000000, 0.000000000000000000 ) ) ;
#69258=ORIENTED_EDGE ( 'NONE', *, *, #39782, .F. ) ;
#69331=ORIENTED_EDGE ( 'NONE', *, *, #64112, .T. ) ;
#69470=ADVANCED_FACE ( 'NONE', ( #43841 ), #64973, .T. ) ;
ENDSEC;
END-ISO-10303-21;
